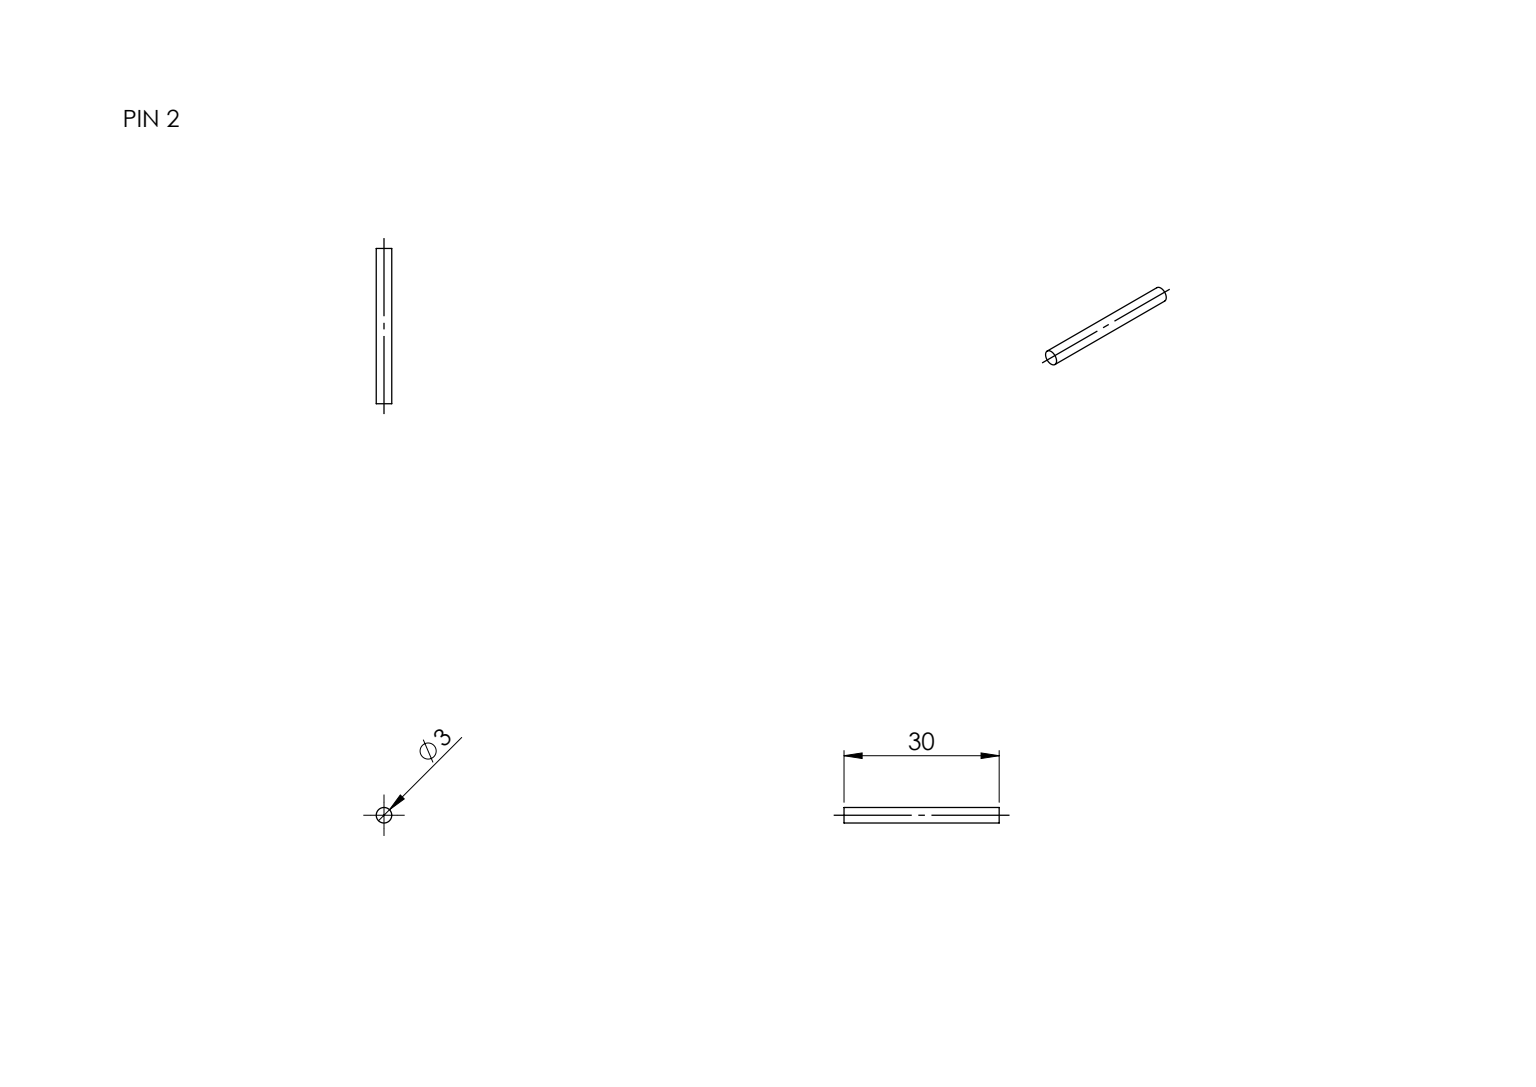
ISO-10303-21;
HEADER;
FILE_DESCRIPTION (('STEP AP214'),
    '1' );
FILE_NAME ('pin 2.step',
    '2026-10-04T07:56:41',
    ( '' ),
    ( '' ),
    'SwSTEP 2.0',
    'SolidWorks 2026',
    '' );
FILE_SCHEMA (( 'AUTOMOTIVE_DESIGN' ));
ENDSEC;

DATA;
#115=AXIS2_PLACEMENT_3D ( 'NONE', #3789, #4326, #6319 ) ;
#130=DIRECTION ( 'NONE',  ( -1.000000000000000000, 0.000000000000000000, 0.000000000000000000 ) ) ;
#153=SHAPE_REPRESENTATION ( 'pin 2', ( #2840 ), #1883 ) ;
#220=SURFACE_SIDE_STYLE ('',( #2333 ) ) ;
#257=DIRECTION ( 'NONE',  ( 0.000000000000000000, 0.000000000000000000, 1.000000000000000000 ) ) ;
#333=PLANE ( 'NONE',  #3355 ) ;
#342=SURFACE_STYLE_USAGE ( .BOTH. , #220 ) ;
#395=CIRCLE ( 'NONE', #1478, 1.499999999999999556 ) ;
#429=( NAMED_UNIT ( * ) SI_UNIT ( $, .STERADIAN. ) SOLID_ANGLE_UNIT ( ) );
#451=MECHANICAL_DESIGN_GEOMETRIC_PRESENTATION_REPRESENTATION('',(#5824),#5564);
#590=DIRECTION ( 'NONE',  ( 1.000000000000000000, 0.000000000000000000, 0.000000000000000000 ) ) ;
#737=DIRECTION ( 'NONE',  ( -1.000000000000000000, 0.000000000000000000, 0.000000000000000000 ) ) ;
#800=CARTESIAN_POINT ( 'NONE',  ( 1.499999999999999556, -9.999999999999994671, -30.00000000000000000 ) ) ;
#844=CARTESIAN_POINT ( 'NONE',  ( 1.499999999999999556, -9.999999999999994671, 0.000000000000000000 ) ) ;
#877=CARTESIAN_POINT ( 'NONE',  ( 0.000000000000000000, -9.999999999999994671, 0.000000000000000000 ) ) ;
#927=ORIENTED_EDGE ( 'NONE', *, *, #4641, .T. ) ;
#1147=EDGE_LOOP ( 'NONE', ( #8081, #927 ) ) ;
#1152=SURFACE_SIDE_STYLE ('',( #2418 ) ) ;
#1309=APPLICATION_CONTEXT ( 'automotive_design' ) ;
#1385=ORIENTED_EDGE ( 'NONE', *, *, #8097, .T. ) ;
#1396=AXIS2_PLACEMENT_3D ( 'NONE', #877, #2027, #3452 ) ;
#1410=ORIENTED_EDGE ( 'NONE', *, *, #4273, .F. ) ;
#1426=EDGE_CURVE ( 'NONE', #4198, #4887, #2956, .T. ) ;
#1478=AXIS2_PLACEMENT_3D ( 'NONE', #7633, #1869, #590 ) ;
#1480=CARTESIAN_POINT ( 'NONE',  ( 0.000000000000000000, -9.999999999999994671, 0.000000000000000000 ) ) ;
#1562=DIRECTION ( 'NONE',  ( 0.000000000000000000, 0.000000000000000000, 1.000000000000000000 ) ) ;
#1585=DIRECTION ( 'NONE',  ( 0.000000000000000000, 0.000000000000000000, 1.000000000000000000 ) ) ;
#1677=ADVANCED_BREP_SHAPE_REPRESENTATION ( '', ( #4428, #2840 ), #1883 ) ;
#1694=DIRECTION ( 'NONE',  ( 1.000000000000000000, 0.000000000000000000, 0.000000000000000000 ) ) ;
#1756=DIRECTION ( 'NONE',  ( 1.000000000000000000, 0.000000000000000000, 0.000000000000000000 ) ) ;
#1801=CIRCLE ( 'NONE', #1396, 1.499999999999999556 ) ;
#1831=PRESENTATION_STYLE_ASSIGNMENT (( #3875 ) ) ;
#1859=PRODUCT_DEFINITION_SHAPE ( 'NONE', 'NONE',  #6847 ) ;
#1869=DIRECTION ( 'NONE',  ( 0.000000000000000000, 0.000000000000000000, 1.000000000000000000 ) ) ;
#1883=( GEOMETRIC_REPRESENTATION_CONTEXT ( 3 ) GLOBAL_UNCERTAINTY_ASSIGNED_CONTEXT ( ( #2253 ) ) GLOBAL_UNIT_ASSIGNED_CONTEXT ( ( #7434, #6205, #429 ) ) REPRESENTATION_CONTEXT ( 'NONE', 'WORKASPACE' ) );
#2027=DIRECTION ( 'NONE',  ( 0.000000000000000000, 0.000000000000000000, 1.000000000000000000 ) ) ;
#2253=UNCERTAINTY_MEASURE_WITH_UNIT (LENGTH_MEASURE( 1.000000000000000082E-05 ), #7434, 'distance_accuracy_value', 'NONE');
#2333=SURFACE_STYLE_FILL_AREA ( #2843 ) ;
#2418=SURFACE_STYLE_FILL_AREA ( #6249 ) ;
#2521=ADVANCED_FACE ( 'NONE', ( #5959 ), #7824, .T. ) ;
#2682=CARTESIAN_POINT ( 'NONE',  ( 0.000000000000000000, -9.999999999999994671, -34.24264068711928388 ) ) ;
#2700=CARTESIAN_POINT ( 'NONE',  ( -1.499999999999999556, -9.999999999999994671, -30.00000000000000000 ) ) ;
#2730=CARTESIAN_POINT ( 'NONE',  ( 1.499999999999999556, -9.999999999999994671, -34.24264068711928388 ) ) ;
#2807=DIRECTION ( 'NONE',  ( 1.000000000000000000, 0.000000000000000000, 0.000000000000000000 ) ) ;
#2840=AXIS2_PLACEMENT_3D ( 'NONE', #8120, #5497, #1756 ) ;
#2842=UNCERTAINTY_MEASURE_WITH_UNIT (LENGTH_MEASURE( 1.000000000000000082E-05 ), #6571, 'distance_accuracy_value', 'NONE');
#2843=FILL_AREA_STYLE ('',( #4810 ) ) ;
#2956=LINE ( 'NONE', #4763, #6693 ) ;
#2961=VECTOR ( 'NONE', #1585, 1000.000000000000000 ) ;
#3047=FILL_AREA_STYLE_COLOUR ( '', #6324 ) ;
#3071=ORIENTED_EDGE ( 'NONE', *, *, #5463, .T. ) ;
#3186=EDGE_LOOP ( 'NONE', ( #3071, #4990, #1410, #7346 ) ) ;
#3355=AXIS2_PLACEMENT_3D ( 'NONE', #1480, #1562, #7252 ) ;
#3424=FACE_OUTER_BOUND ( 'NONE', #3186, .T. ) ;
#3452=DIRECTION ( 'NONE',  ( 1.000000000000000000, 0.000000000000000000, 0.000000000000000000 ) ) ;
#3589=( NAMED_UNIT ( * ) SI_UNIT ( $, .STERADIAN. ) SOLID_ANGLE_UNIT ( ) );
#3627=STYLED_ITEM ( 'NONE', ( #1831 ), #1677 ) ;
#3758=ORIENTED_EDGE ( 'NONE', *, *, #4641, .F. ) ;
#3788=EDGE_LOOP ( 'NONE', ( #6885, #5797, #1385, #3758 ) ) ;
#3789=CARTESIAN_POINT ( 'NONE',  ( 0.000000000000000000, -9.999999999999994671, -30.00000000000000000 ) ) ;
#3875=SURFACE_STYLE_USAGE ( .BOTH. , #1152 ) ;
#4007=PLANE ( 'NONE',  #7537 ) ;
#4057=( NAMED_UNIT ( * ) PLANE_ANGLE_UNIT ( ) SI_UNIT ( $, .RADIAN. ) );
#4090=DIRECTION ( 'NONE',  ( 0.000000000000000000, 0.000000000000000000, 1.000000000000000000 ) ) ;
#4168=FACE_OUTER_BOUND ( 'NONE', #1147, .T. ) ;
#4198=VERTEX_POINT ( 'NONE', #2700 ) ;
#4205=PRODUCT_CONTEXT ( 'NONE', #5020, 'mechanical' ) ;
#4216=COLOUR_RGB ( '', 0.40784314, 0.44705882, 0.49803922) ;
#4273=EDGE_CURVE ( 'NONE', #5032, #4887, #1801, .T. ) ;
#4326=DIRECTION ( 'NONE',  ( -0.000000000000000000, -0.000000000000000000, 1.000000000000000000 ) ) ;
#4428=MANIFOLD_SOLID_BREP ( 'Boss-Extrude1', #5039 ) ;
#4564=CARTESIAN_POINT ( 'NONE',  ( 0.000000000000000000, -9.999999999999994671, -30.00000000000000000 ) ) ;
#4605=DIRECTION ( 'NONE',  ( -0.000000000000000000, -0.000000000000000000, 1.000000000000000000 ) ) ;
#4641=EDGE_CURVE ( 'NONE', #4887, #5032, #395, .T. ) ;
#4701=AXIS2_PLACEMENT_3D ( 'NONE', #4564, #4605, #737 ) ;
#4730=DIRECTION ( 'NONE',  ( 0.000000000000000000, 0.000000000000000000, 1.000000000000000000 ) ) ;
#4763=CARTESIAN_POINT ( 'NONE',  ( -1.499999999999999556, -9.999999999999994671, -34.24264068711928388 ) ) ;
#4810=FILL_AREA_STYLE_COLOUR ( '', #4216 ) ;
#4811=VERTEX_POINT ( 'NONE', #800 ) ;
#4843=SHAPE_DEFINITION_REPRESENTATION ( #1859, #153 ) ;
#4857=( LENGTH_UNIT ( ) NAMED_UNIT ( * ) SI_UNIT ( .MILLI., .METRE. ) );
#4875=PRODUCT ( 'pin 2', 'pin 2', '', ( #4205 ) ) ;
#4887=VERTEX_POINT ( 'NONE', #6575 ) ;
#4969=( GEOMETRIC_REPRESENTATION_CONTEXT ( 3 ) GLOBAL_UNCERTAINTY_ASSIGNED_CONTEXT ( ( #2842 ) ) GLOBAL_UNIT_ASSIGNED_CONTEXT ( ( #6571, #6444, #7758 ) ) REPRESENTATION_CONTEXT ( 'NONE', 'WORKASPACE' ) );
#4990=ORIENTED_EDGE ( 'NONE', *, *, #1426, .T. ) ;
#5020=APPLICATION_CONTEXT ( 'automotive_design' ) ;
#5032=VERTEX_POINT ( 'NONE', #844 ) ;
#5039=CLOSED_SHELL ( 'NONE', ( #7731, #7441, #5065, #2521 ) ) ;
#5065=ADVANCED_FACE ( 'NONE', ( #4168 ), #333, .T. ) ;
#5099=MECHANICAL_DESIGN_GEOMETRIC_PRESENTATION_REPRESENTATION('',(#3627),#4969);
#5368=CIRCLE ( 'NONE', #115, 1.499999999999999556 ) ;
#5402=ORIENTED_EDGE ( 'NONE', *, *, #5463, .F. ) ;
#5463=EDGE_CURVE ( 'NONE', #4811, #4198, #5368, .T. ) ;
#5497=DIRECTION ( 'NONE',  ( 0.000000000000000000, 0.000000000000000000, 1.000000000000000000 ) ) ;
#5512=AXIS2_PLACEMENT_3D ( 'NONE', #8101, #4090, #1694 ) ;
#5564=( GEOMETRIC_REPRESENTATION_CONTEXT ( 3 ) GLOBAL_UNCERTAINTY_ASSIGNED_CONTEXT ( ( #8160 ) ) GLOBAL_UNIT_ASSIGNED_CONTEXT ( ( #4857, #4057, #3589 ) ) REPRESENTATION_CONTEXT ( 'NONE', 'WORKASPACE' ) );
#5617=EDGE_LOOP ( 'NONE', ( #5402, #6687 ) ) ;
#5797=ORIENTED_EDGE ( 'NONE', *, *, #8014, .T. ) ;
#5824=STYLED_ITEM ( 'NONE', ( #7385 ), #4428 ) ;
#5959=FACE_OUTER_BOUND ( 'NONE', #3788, .T. ) ;
#6028=CYLINDRICAL_SURFACE ( 'NONE', #5512, 1.499999999999999556 ) ;
#6205=( NAMED_UNIT ( * ) PLANE_ANGLE_UNIT ( ) SI_UNIT ( $, .RADIAN. ) );
#6241=AXIS2_PLACEMENT_3D ( 'NONE', #2682, #4730, #2807 ) ;
#6249=FILL_AREA_STYLE ('',( #3047 ) ) ;
#6314=PRODUCT_DEFINITION_FORMATION_WITH_SPECIFIED_SOURCE ( 'ANY', '', #4875, .NOT_KNOWN. ) ;
#6319=DIRECTION ( 'NONE',  ( -1.000000000000000000, 0.000000000000000000, 0.000000000000000000 ) ) ;
#6324=COLOUR_RGB ( '', 0.40784314, 0.44705882, 0.49803922) ;
#6444=( NAMED_UNIT ( * ) PLANE_ANGLE_UNIT ( ) SI_UNIT ( $, .RADIAN. ) );
#6571=( LENGTH_UNIT ( ) NAMED_UNIT ( * ) SI_UNIT ( .MILLI., .METRE. ) );
#6575=CARTESIAN_POINT ( 'NONE',  ( -1.499999999999999556, -9.999999999999994671, 0.000000000000000000 ) ) ;
#6592=CIRCLE ( 'NONE', #4701, 1.499999999999999556 ) ;
#6687=ORIENTED_EDGE ( 'NONE', *, *, #8014, .F. ) ;
#6693=VECTOR ( 'NONE', #257, 1000.000000000000000 ) ;
#6847=PRODUCT_DEFINITION ( 'UNKNOWN', '', #6314, #7384 ) ;
#6885=ORIENTED_EDGE ( 'NONE', *, *, #1426, .F. ) ;
#6959=SHAPE_REPRESENTATION_RELATIONSHIP ( 'NONE' , 'NONE' ,  #153, #1677 ) ;
#7084=FACE_OUTER_BOUND ( 'NONE', #5617, .T. ) ;
#7233=LINE ( 'NONE', #2730, #2961 ) ;
#7252=DIRECTION ( 'NONE',  ( 1.000000000000000000, 0.000000000000000000, -0.000000000000000000 ) ) ;
#7346=ORIENTED_EDGE ( 'NONE', *, *, #8097, .F. ) ;
#7384=PRODUCT_DEFINITION_CONTEXT ( 'detailed design', #1309, 'design' ) ;
#7385=PRESENTATION_STYLE_ASSIGNMENT (( #342 ) ) ;
#7434=( LENGTH_UNIT ( ) NAMED_UNIT ( * ) SI_UNIT ( .MILLI., .METRE. ) );
#7441=ADVANCED_FACE ( 'NONE', ( #7084 ), #4007, .T. ) ;
#7537=AXIS2_PLACEMENT_3D ( 'NONE', #7764, #7851, #130 ) ;
#7633=CARTESIAN_POINT ( 'NONE',  ( 0.000000000000000000, -9.999999999999994671, 0.000000000000000000 ) ) ;
#7731=ADVANCED_FACE ( 'NONE', ( #3424 ), #6028, .T. ) ;
#7758=( NAMED_UNIT ( * ) SI_UNIT ( $, .STERADIAN. ) SOLID_ANGLE_UNIT ( ) );
#7764=CARTESIAN_POINT ( 'NONE',  ( 0.000000000000000000, 0.000000000000000000, -30.00000000000000000 ) ) ;
#7824=CYLINDRICAL_SURFACE ( 'NONE', #6241, 1.499999999999999556 ) ;
#7851=DIRECTION ( 'NONE',  ( 0.000000000000000000, 0.000000000000000000, -1.000000000000000000 ) ) ;
#8014=EDGE_CURVE ( 'NONE', #4198, #4811, #6592, .T. ) ;
#8081=ORIENTED_EDGE ( 'NONE', *, *, #4273, .T. ) ;
#8097=EDGE_CURVE ( 'NONE', #4811, #5032, #7233, .T. ) ;
#8101=CARTESIAN_POINT ( 'NONE',  ( 0.000000000000000000, -9.999999999999994671, -34.24264068711928388 ) ) ;
#8120=CARTESIAN_POINT ( 'NONE',  ( 0.000000000000000000, 0.000000000000000000, 0.000000000000000000 ) ) ;
#8160=UNCERTAINTY_MEASURE_WITH_UNIT (LENGTH_MEASURE( 1.000000000000000082E-05 ), #4857, 'distance_accuracy_value', 'NONE');
ENDSEC;
END-ISO-10303-21;
